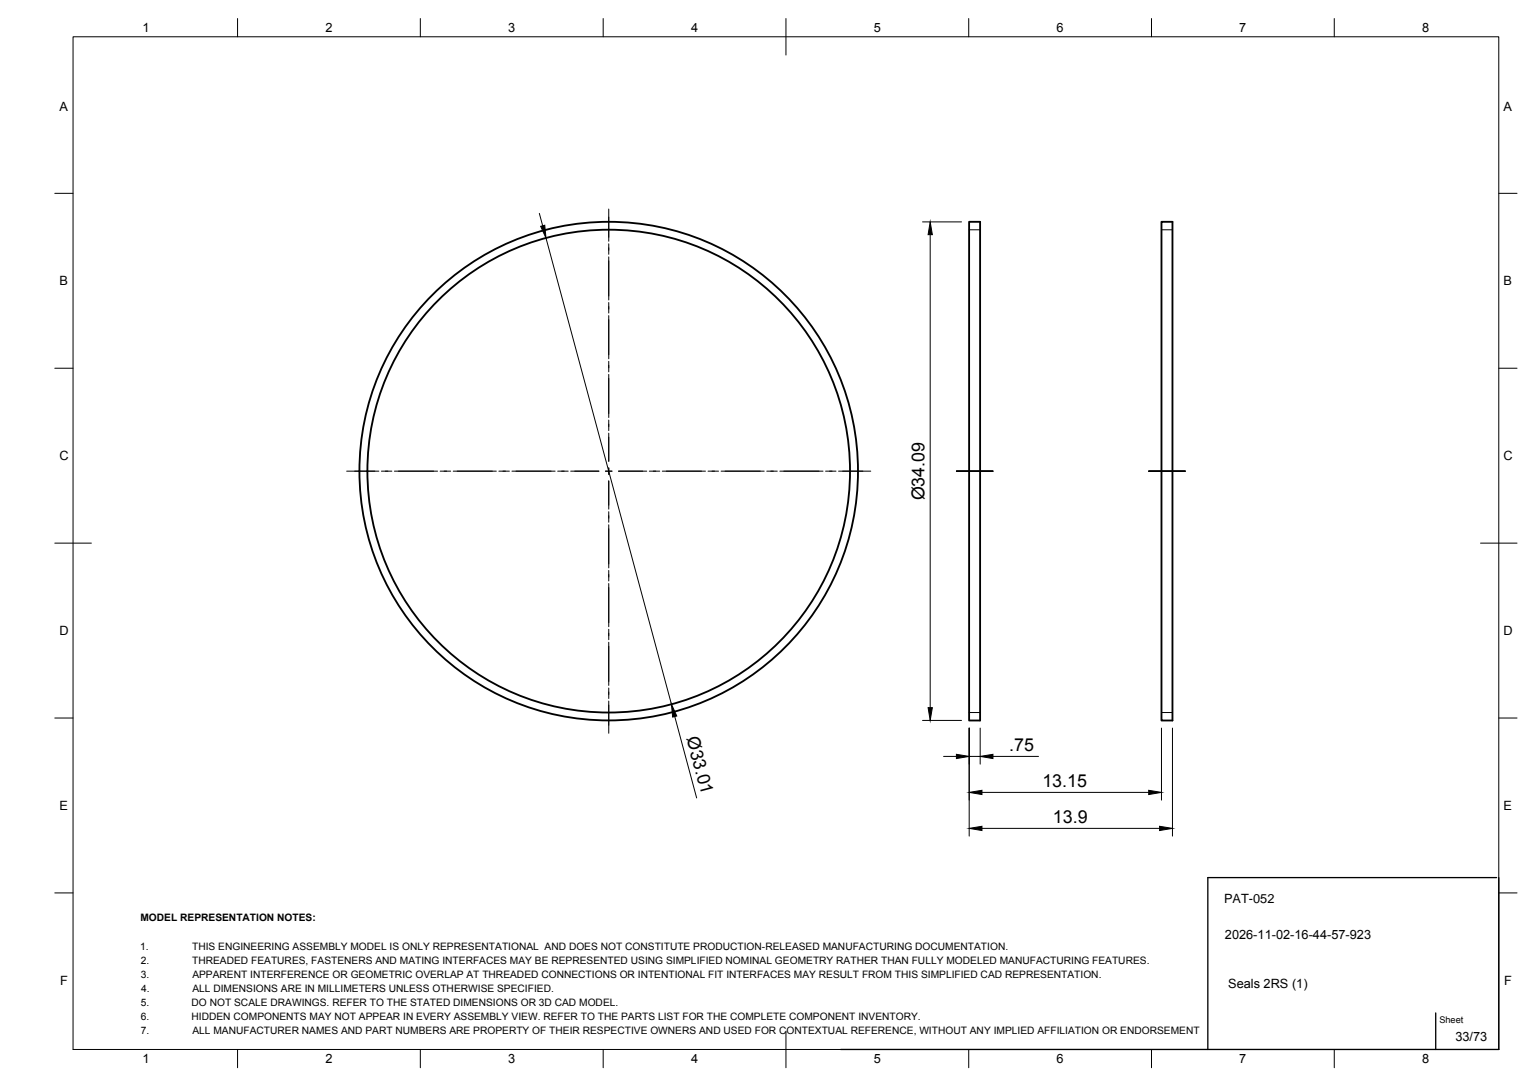
ISO-10303-21;
HEADER;
/* Generated by software containing ST-Developer
 * from STEP Tools, Inc. (www.steptools.com) 
 */

FILE_DESCRIPTION(
/* description */ ('Hand-crank gear train demonstrator'),
/* implementation_level */ '2;1');

FILE_NAME(
/* name */ 'Seals 2RS (1).step',
/* time_stamp */ '2026-10-28T03:22:13-07:00',
/* author */ (''),
/* organization */ (''),
/* preprocessor_version */ 'ST-DEVELOPER v20.2',
/* originating_system */ 'Autodesk Translation Framework v15.17.0.0',
/* authorisation */ '');

FILE_SCHEMA (('AUTOMOTIVE_DESIGN { 1 0 10303 214 3 1 1 }'));
ENDSEC;

DATA;
#10=MECHANICAL_DESIGN_GEOMETRIC_PRESENTATION_REPRESENTATION('',(#1223,#1224),#62758);
#1081=SHAPE_REPRESENTATION_RELATIONSHIP('SRR','None',#63055,#1145);
#1145=ADVANCED_BREP_SHAPE_REPRESENTATION('',(#1301,#1302),#62709);
#1223=STYLED_ITEM('',(#63462),#1301);
#1224=STYLED_ITEM('',(#63462),#1302);
#1301=MANIFOLD_SOLID_BREP('Body1',#16404);
#1302=MANIFOLD_SOLID_BREP('Body2',#16405);
#1501=FACE_BOUND('',#3448,.T.);
#1502=FACE_BOUND('',#3451,.T.);
#1503=FACE_BOUND('',#3454,.T.);
#1504=FACE_BOUND('',#3457,.T.);
#1711=PLANE('',#17725);
#1712=PLANE('',#17730);
#1713=PLANE('',#17733);
#1714=PLANE('',#17738);
#2352=FACE_OUTER_BOUND('',#3447,.T.);
#2353=FACE_OUTER_BOUND('',#3449,.T.);
#2354=FACE_OUTER_BOUND('',#3450,.T.);
#2355=FACE_OUTER_BOUND('',#3452,.T.);
#2356=FACE_OUTER_BOUND('',#3453,.T.);
#2357=FACE_OUTER_BOUND('',#3455,.T.);
#2358=FACE_OUTER_BOUND('',#3456,.T.);
#2359=FACE_OUTER_BOUND('',#3458,.T.);
#3447=EDGE_LOOP('',(#11845));
#3448=EDGE_LOOP('',(#11846));
#3449=EDGE_LOOP('',(#11847,#11848,#11849,#11850));
#3450=EDGE_LOOP('',(#11851));
#3451=EDGE_LOOP('',(#11852));
#3452=EDGE_LOOP('',(#11853,#11854,#11855,#11856));
#3453=EDGE_LOOP('',(#11857));
#3454=EDGE_LOOP('',(#11858));
#3455=EDGE_LOOP('',(#11859,#11860,#11861,#11862));
#3456=EDGE_LOOP('',(#11863));
#3457=EDGE_LOOP('',(#11864));
#3458=EDGE_LOOP('',(#11865,#11866,#11867,#11868));
#4451=LINE('',#25066,#5583);
#4452=LINE('',#25071,#5584);
#4453=LINE('',#25080,#5585);
#4454=LINE('',#25085,#5586);
#5583=VECTOR('',#20140,1.70469);
#5584=VECTOR('',#20147,1.65031);
#5585=VECTOR('',#20158,1.70469);
#5586=VECTOR('',#20165,1.65031);
#6858=CIRCLE('',#17726,1.70469);
#6859=CIRCLE('',#17727,1.65031);
#6860=CIRCLE('',#17729,1.70469);
#6861=CIRCLE('',#17731,1.65031);
#6862=CIRCLE('',#17734,1.70469);
#6863=CIRCLE('',#17735,1.65031);
#6864=CIRCLE('',#17737,1.70469);
#6865=CIRCLE('',#17739,1.65031);
#7565=VERTEX_POINT('',#25059);
#7566=VERTEX_POINT('',#25061);
#7567=VERTEX_POINT('',#25064);
#7568=VERTEX_POINT('',#25068);
#7569=VERTEX_POINT('',#25073);
#7570=VERTEX_POINT('',#25075);
#7571=VERTEX_POINT('',#25078);
#7572=VERTEX_POINT('',#25082);
#9174=EDGE_CURVE('',#7565,#7565,#6858,.T.);
#9175=EDGE_CURVE('',#7566,#7566,#6859,.T.);
#9176=EDGE_CURVE('',#7567,#7567,#6860,.T.);
#9177=EDGE_CURVE('',#7567,#7565,#4451,.T.);
#9178=EDGE_CURVE('',#7568,#7568,#6861,.T.);
#9179=EDGE_CURVE('',#7568,#7566,#4452,.T.);
#9180=EDGE_CURVE('',#7569,#7569,#6862,.T.);
#9181=EDGE_CURVE('',#7570,#7570,#6863,.T.);
#9182=EDGE_CURVE('',#7571,#7571,#6864,.T.);
#9183=EDGE_CURVE('',#7571,#7569,#4453,.T.);
#9184=EDGE_CURVE('',#7572,#7572,#6865,.T.);
#9185=EDGE_CURVE('',#7572,#7570,#4454,.T.);
#11845=ORIENTED_EDGE('',*,*,#9174,.F.);
#11846=ORIENTED_EDGE('',*,*,#9175,.T.);
#11847=ORIENTED_EDGE('',*,*,#9176,.F.);
#11848=ORIENTED_EDGE('',*,*,#9177,.T.);
#11849=ORIENTED_EDGE('',*,*,#9174,.T.);
#11850=ORIENTED_EDGE('',*,*,#9177,.F.);
#11851=ORIENTED_EDGE('',*,*,#9176,.T.);
#11852=ORIENTED_EDGE('',*,*,#9178,.F.);
#11853=ORIENTED_EDGE('',*,*,#9178,.T.);
#11854=ORIENTED_EDGE('',*,*,#9179,.T.);
#11855=ORIENTED_EDGE('',*,*,#9175,.F.);
#11856=ORIENTED_EDGE('',*,*,#9179,.F.);
#11857=ORIENTED_EDGE('',*,*,#9180,.F.);
#11858=ORIENTED_EDGE('',*,*,#9181,.T.);
#11859=ORIENTED_EDGE('',*,*,#9182,.F.);
#11860=ORIENTED_EDGE('',*,*,#9183,.T.);
#11861=ORIENTED_EDGE('',*,*,#9180,.T.);
#11862=ORIENTED_EDGE('',*,*,#9183,.F.);
#11863=ORIENTED_EDGE('',*,*,#9182,.T.);
#11864=ORIENTED_EDGE('',*,*,#9184,.F.);
#11865=ORIENTED_EDGE('',*,*,#9184,.T.);
#11866=ORIENTED_EDGE('',*,*,#9185,.T.);
#11867=ORIENTED_EDGE('',*,*,#9181,.F.);
#11868=ORIENTED_EDGE('',*,*,#9185,.F.);
#15273=CYLINDRICAL_SURFACE('',#17728,1.70469);
#15274=CYLINDRICAL_SURFACE('',#17732,1.65031);
#15275=CYLINDRICAL_SURFACE('',#17736,1.70469);
#15276=CYLINDRICAL_SURFACE('',#17740,1.65031);
#15662=ADVANCED_FACE('',(#2352,#1501),#1711,.T.);
#15663=ADVANCED_FACE('',(#2353),#15273,.T.);
#15664=ADVANCED_FACE('',(#2354,#1502),#1712,.T.);
#15665=ADVANCED_FACE('',(#2355),#15274,.F.);
#15666=ADVANCED_FACE('',(#2356,#1503),#1713,.T.);
#15667=ADVANCED_FACE('',(#2357),#15275,.T.);
#15668=ADVANCED_FACE('',(#2358,#1504),#1714,.T.);
#15669=ADVANCED_FACE('',(#2359),#15276,.F.);
#16404=CLOSED_SHELL('',(#15662,#15663,#15664,#15665));
#16405=CLOSED_SHELL('',(#15666,#15667,#15668,#15669));
#17724=AXIS2_PLACEMENT_3D('',#25057,#20128,#20129);
#17725=AXIS2_PLACEMENT_3D('',#25058,#20130,#20131);
#17726=AXIS2_PLACEMENT_3D('',#25060,#20132,#20133);
#17727=AXIS2_PLACEMENT_3D('',#25062,#20134,#20135);
#17728=AXIS2_PLACEMENT_3D('',#25063,#20136,#20137);
#17729=AXIS2_PLACEMENT_3D('',#25065,#20138,#20139);
#17730=AXIS2_PLACEMENT_3D('',#25067,#20141,#20142);
#17731=AXIS2_PLACEMENT_3D('',#25069,#20143,#20144);
#17732=AXIS2_PLACEMENT_3D('',#25070,#20145,#20146);
#17733=AXIS2_PLACEMENT_3D('',#25072,#20148,#20149);
#17734=AXIS2_PLACEMENT_3D('',#25074,#20150,#20151);
#17735=AXIS2_PLACEMENT_3D('',#25076,#20152,#20153);
#17736=AXIS2_PLACEMENT_3D('',#25077,#20154,#20155);
#17737=AXIS2_PLACEMENT_3D('',#25079,#20156,#20157);
#17738=AXIS2_PLACEMENT_3D('',#25081,#20159,#20160);
#17739=AXIS2_PLACEMENT_3D('',#25083,#20161,#20162);
#17740=AXIS2_PLACEMENT_3D('',#25084,#20163,#20164);
#20128=DIRECTION('axis',(0.,0.,1.));
#20129=DIRECTION('refdir',(1.,0.,0.));
#20130=DIRECTION('center_axis',(0.,1.,0.));
#20131=DIRECTION('ref_axis',(0.,0.,1.));
#20132=DIRECTION('center_axis',(0.,-1.,0.));
#20133=DIRECTION('ref_axis',(1.,0.,0.));
#20134=DIRECTION('center_axis',(0.,-1.,0.));
#20135=DIRECTION('ref_axis',(1.,0.,0.));
#20136=DIRECTION('center_axis',(0.,-1.,0.));
#20137=DIRECTION('ref_axis',(1.,0.,0.));
#20138=DIRECTION('center_axis',(0.,-1.,0.));
#20139=DIRECTION('ref_axis',(1.,0.,0.));
#20140=DIRECTION('',(0.,1.,0.));
#20141=DIRECTION('center_axis',(0.,-1.,0.));
#20142=DIRECTION('ref_axis',(0.,0.,-1.));
#20143=DIRECTION('center_axis',(0.,-1.,0.));
#20144=DIRECTION('ref_axis',(1.,0.,0.));
#20145=DIRECTION('center_axis',(0.,-1.,0.));
#20146=DIRECTION('ref_axis',(1.,0.,0.));
#20147=DIRECTION('',(0.,1.,0.));
#20148=DIRECTION('center_axis',(0.,1.,0.));
#20149=DIRECTION('ref_axis',(0.,0.,1.));
#20150=DIRECTION('center_axis',(0.,-1.,0.));
#20151=DIRECTION('ref_axis',(1.,0.,0.));
#20152=DIRECTION('center_axis',(0.,-1.,0.));
#20153=DIRECTION('ref_axis',(1.,0.,0.));
#20154=DIRECTION('center_axis',(0.,-1.,0.));
#20155=DIRECTION('ref_axis',(1.,0.,0.));
#20156=DIRECTION('center_axis',(0.,-1.,0.));
#20157=DIRECTION('ref_axis',(1.,0.,0.));
#20158=DIRECTION('',(0.,1.,0.));
#20159=DIRECTION('center_axis',(0.,-1.,0.));
#20160=DIRECTION('ref_axis',(0.,0.,-1.));
#20161=DIRECTION('center_axis',(0.,-1.,0.));
#20162=DIRECTION('ref_axis',(1.,0.,0.));
#20163=DIRECTION('center_axis',(0.,-1.,0.));
#20164=DIRECTION('ref_axis',(1.,0.,0.));
#20165=DIRECTION('',(0.,1.,0.));
#25057=CARTESIAN_POINT('',(0.,0.,0.));
#25058=CARTESIAN_POINT('Origin',(1.70469,0.695,0.));
#25059=CARTESIAN_POINT('',(-1.70469,0.695,-2.0876431520385E-16));
#25060=CARTESIAN_POINT('Origin',(0.,0.695,0.));
#25061=CARTESIAN_POINT('',(-1.65031,0.695,-2.02104685910087E-16));
#25062=CARTESIAN_POINT('Origin',(0.,0.695,0.));
#25063=CARTESIAN_POINT('Origin',(0.,0.6575,0.));
#25064=CARTESIAN_POINT('',(-1.70469,0.62,-2.0876431520385E-16));
#25065=CARTESIAN_POINT('Origin',(0.,0.62,0.));
#25066=CARTESIAN_POINT('',(-1.70469,0.6575,-2.0876431520385E-16));
#25067=CARTESIAN_POINT('Origin',(1.65031,0.62,0.));
#25068=CARTESIAN_POINT('',(-1.65031,0.62,-2.02104685910087E-16));
#25069=CARTESIAN_POINT('Origin',(0.,0.62,0.));
#25070=CARTESIAN_POINT('Origin',(0.,0.6575,0.));
#25071=CARTESIAN_POINT('',(-1.65031,0.6575,-2.02104685910087E-16));
#25072=CARTESIAN_POINT('Origin',(1.70469,-0.62,0.));
#25073=CARTESIAN_POINT('',(-1.70469,-0.62,-2.0876431520385E-16));
#25074=CARTESIAN_POINT('Origin',(0.,-0.62,0.));
#25075=CARTESIAN_POINT('',(-1.65031,-0.62,-2.02104685910087E-16));
#25076=CARTESIAN_POINT('Origin',(0.,-0.62,0.));
#25077=CARTESIAN_POINT('Origin',(0.,-0.6575,0.));
#25078=CARTESIAN_POINT('',(-1.70469,-0.695,-2.0876431520385E-16));
#25079=CARTESIAN_POINT('Origin',(0.,-0.695,0.));
#25080=CARTESIAN_POINT('',(-1.70469,-0.6575,-2.0876431520385E-16));
#25081=CARTESIAN_POINT('Origin',(1.65031,-0.695,0.));
#25082=CARTESIAN_POINT('',(-1.65031,-0.695,-2.02104685910087E-16));
#25083=CARTESIAN_POINT('Origin',(0.,-0.695,0.));
#25084=CARTESIAN_POINT('Origin',(0.,-0.6575,0.));
#25085=CARTESIAN_POINT('',(-1.65031,-0.6575,-2.02104685910087E-16));
#62635=UNCERTAINTY_MEASURE_WITH_UNIT(LENGTH_MEASURE(0.001),#62759,
'DISTANCE_ACCURACY_VALUE',
'Maximum model space distance between geometric entities at asserted c
onnectivities');
#62684=UNCERTAINTY_MEASURE_WITH_UNIT(LENGTH_MEASURE(0.001),#62759,
'DISTANCE_ACCURACY_VALUE',
'Maximum model space distance between geometric entities at asserted c
onnectivities');
#62709=(
GEOMETRIC_REPRESENTATION_CONTEXT(3)
GLOBAL_UNCERTAINTY_ASSIGNED_CONTEXT((#62635))
GLOBAL_UNIT_ASSIGNED_CONTEXT((#62759,#62761,#62762))
REPRESENTATION_CONTEXT('','3D')
);
#62758=(
GEOMETRIC_REPRESENTATION_CONTEXT(3)
GLOBAL_UNCERTAINTY_ASSIGNED_CONTEXT((#62684))
GLOBAL_UNIT_ASSIGNED_CONTEXT((#62759,#62761,#62762))
REPRESENTATION_CONTEXT('','3D')
);
#62759=(
LENGTH_UNIT()
NAMED_UNIT(*)
SI_UNIT(.CENTI.,.METRE.)
);
#62761=(
NAMED_UNIT(*)
PLANE_ANGLE_UNIT()
SI_UNIT($,.RADIAN.)
);
#62762=(
NAMED_UNIT(*)
SI_UNIT($,.STERADIAN.)
SOLID_ANGLE_UNIT()
);
#62787=SHAPE_DEFINITION_REPRESENTATION(#62865,#63055);
#62865=PRODUCT_DEFINITION_SHAPE('',$,#63129);
#63055=SHAPE_REPRESENTATION('',(#17724),#62709);
#63104=PRODUCT_DEFINITION_CONTEXT('part definition',#63325,'design');
#63129=PRODUCT_DEFINITION('Seals 2RS (1)','Seals 2RS (1)',#63202,#63104);
#63202=PRODUCT_DEFINITION_FORMATION('',$,#63351);
#63325=APPLICATION_CONTEXT(
'Core Data for Automotive Mechanical Design Process');
#63326=PRODUCT_CONTEXT('part definition',#63325,'mechanical');
#63351=PRODUCT('Seals 2RS (1)','Seals 2RS (1)','Seals 2RS (1)',(#63326));
#63456=COLOUR_RGB('Grey',0.48,0.52,0.57);
#63457=FILL_AREA_STYLE_COLOUR('',#63456);
#63458=FILL_AREA_STYLE('',(#63457));
#63459=SURFACE_STYLE_FILL_AREA(#63458);
#63460=SURFACE_SIDE_STYLE('',(#63459));
#63461=SURFACE_STYLE_USAGE(.BOTH.,#63460);
#63462=PRESENTATION_STYLE_ASSIGNMENT((#63461));
ENDSEC;
END-ISO-10303-21;
